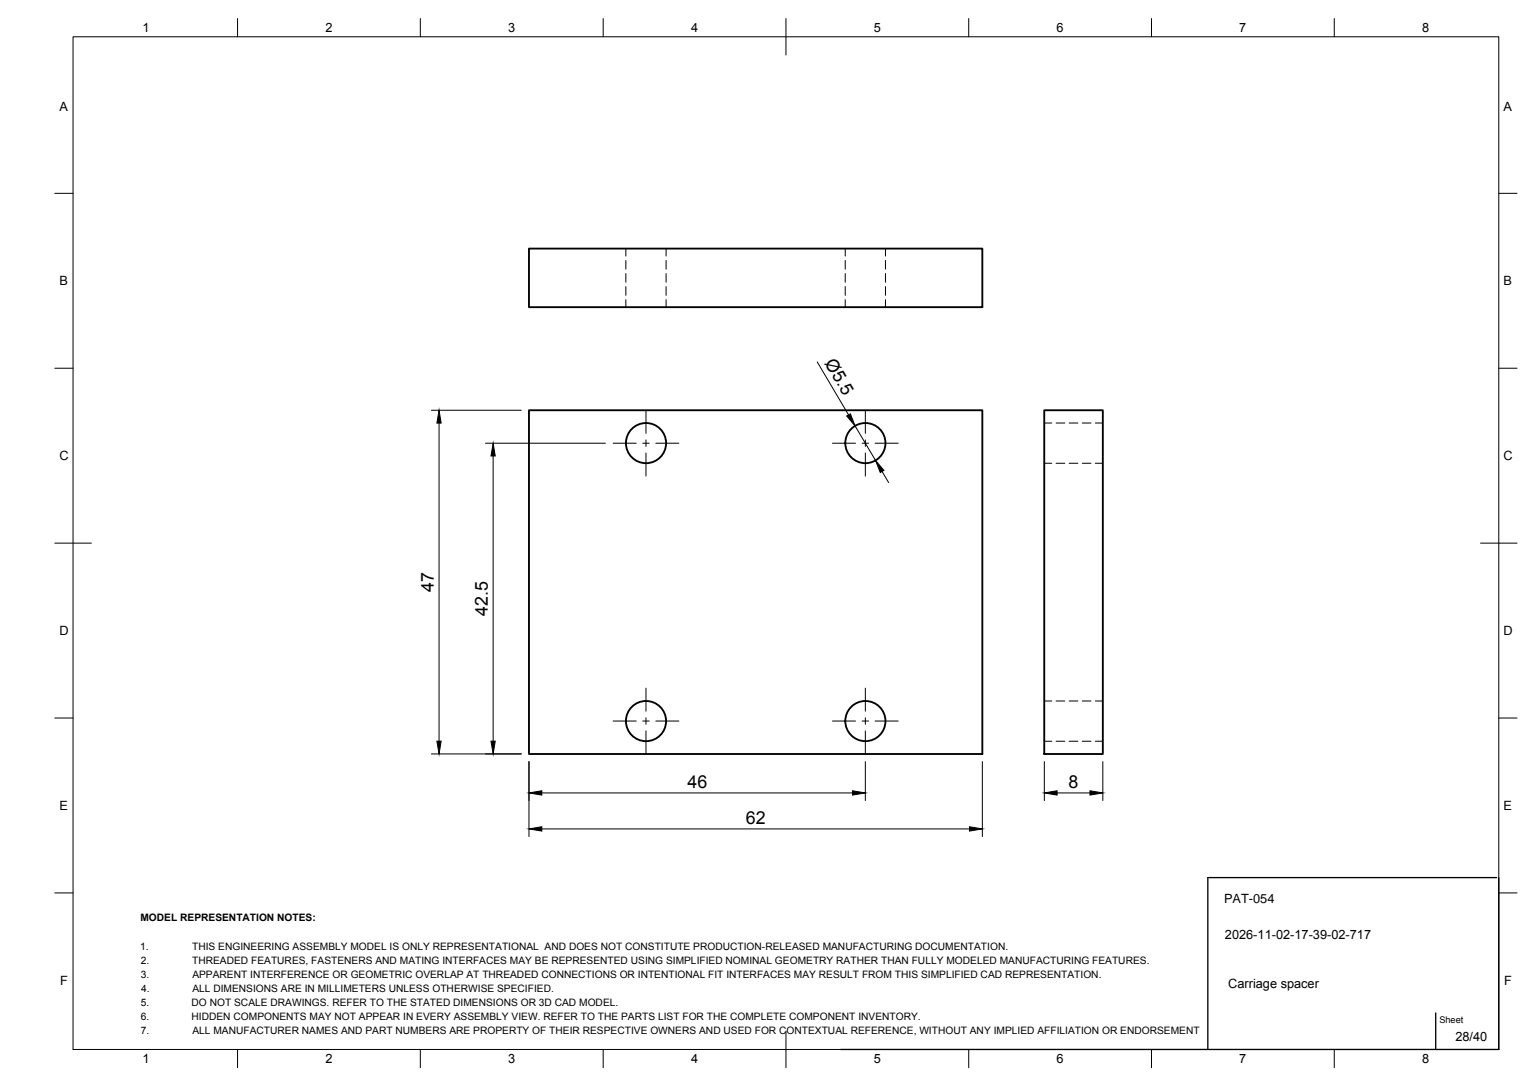
ISO-10303-21;
HEADER;
/* Generated by software containing ST-Developer
 * from STEP Tools, Inc. (www.steptools.com) 
 */

FILE_DESCRIPTION(
/* description */ ('PAT-054'),
/* implementation_level */ '2;1');

FILE_NAME(
/* name */ 'Carriage spacer.step',
/* time_stamp */ '2026-10-29T16:38:13-07:00',
/* author */ (''),
/* organization */ (''),
/* preprocessor_version */ 'ST-DEVELOPER v20.2',
/* originating_system */ 'Autodesk Translation Framework v15.17.0.0',
/* authorisation */ '');

FILE_SCHEMA (('AUTOMOTIVE_DESIGN { 1 0 10303 214 3 1 1 }'));
ENDSEC;

DATA;
#10=MECHANICAL_DESIGN_GEOMETRIC_PRESENTATION_REPRESENTATION('',(#937),#33981);
#834=SHAPE_REPRESENTATION_RELATIONSHIP('SRR','None',#34210,#878);
#878=ADVANCED_BREP_SHAPE_REPRESENTATION('',(#995),#33958);
#937=STYLED_ITEM('',(#34510),#995);
#995=MANIFOLD_SOLID_BREP('Body1',#13049);
#1152=FACE_BOUND('',#2777,.T.);
#1153=FACE_BOUND('',#2778,.T.);
#1154=FACE_BOUND('',#2779,.T.);
#1155=FACE_BOUND('',#2780,.T.);
#1156=FACE_BOUND('',#2782,.T.);
#1157=FACE_BOUND('',#2783,.T.);
#1158=FACE_BOUND('',#2784,.T.);
#1159=FACE_BOUND('',#2785,.T.);
#1412=PLANE('',#14249);
#1413=PLANE('',#14250);
#1414=PLANE('',#14251);
#1415=PLANE('',#14252);
#1416=PLANE('',#14253);
#1417=PLANE('',#14254);
#1905=FACE_OUTER_BOUND('',#2768,.T.);
#1906=FACE_OUTER_BOUND('',#2769,.T.);
#1907=FACE_OUTER_BOUND('',#2770,.T.);
#1908=FACE_OUTER_BOUND('',#2771,.T.);
#1909=FACE_OUTER_BOUND('',#2772,.T.);
#1910=FACE_OUTER_BOUND('',#2773,.T.);
#1911=FACE_OUTER_BOUND('',#2774,.T.);
#1912=FACE_OUTER_BOUND('',#2775,.T.);
#1913=FACE_OUTER_BOUND('',#2776,.T.);
#1914=FACE_OUTER_BOUND('',#2781,.T.);
#2768=EDGE_LOOP('',(#10037,#10038,#10039,#10040));
#2769=EDGE_LOOP('',(#10041,#10042,#10043,#10044));
#2770=EDGE_LOOP('',(#10045,#10046,#10047,#10048));
#2771=EDGE_LOOP('',(#10049,#10050,#10051,#10052));
#2772=EDGE_LOOP('',(#10053,#10054,#10055,#10056));
#2773=EDGE_LOOP('',(#10057,#10058,#10059,#10060));
#2774=EDGE_LOOP('',(#10061,#10062,#10063,#10064));
#2775=EDGE_LOOP('',(#10065,#10066,#10067,#10068));
#2776=EDGE_LOOP('',(#10069,#10070,#10071,#10072));
#2777=EDGE_LOOP('',(#10073));
#2778=EDGE_LOOP('',(#10074));
#2779=EDGE_LOOP('',(#10075));
#2780=EDGE_LOOP('',(#10076));
#2781=EDGE_LOOP('',(#10077,#10078,#10079,#10080));
#2782=EDGE_LOOP('',(#10081));
#2783=EDGE_LOOP('',(#10082));
#2784=EDGE_LOOP('',(#10083));
#2785=EDGE_LOOP('',(#10084));
#3670=LINE('',#20797,#4604);
#3671=LINE('',#20803,#4605);
#3672=LINE('',#20809,#4606);
#3673=LINE('',#20815,#4607);
#3674=LINE('',#20820,#4608);
#3675=LINE('',#20822,#4609);
#3676=LINE('',#20824,#4610);
#3677=LINE('',#20825,#4611);
#3678=LINE('',#20828,#4612);
#3679=LINE('',#20830,#4613);
#3680=LINE('',#20831,#4614);
#3681=LINE('',#20834,#4615);
#3682=LINE('',#20836,#4616);
#3683=LINE('',#20837,#4617);
#3684=LINE('',#20839,#4618);
#3685=LINE('',#20840,#4619);
#4604=VECTOR('',#16683,0.275);
#4605=VECTOR('',#16690,0.275);
#4606=VECTOR('',#16697,0.275);
#4607=VECTOR('',#16704,0.275);
#4608=VECTOR('',#16709,1.);
#4609=VECTOR('',#16710,1.);
#4610=VECTOR('',#16711,1.);
#4611=VECTOR('',#16712,1.);
#4612=VECTOR('',#16715,1.);
#4613=VECTOR('',#16716,1.);
#4614=VECTOR('',#16717,1.);
#4615=VECTOR('',#16720,1.);
#4616=VECTOR('',#16721,1.);
#4617=VECTOR('',#16722,1.);
#4618=VECTOR('',#16725,1.);
#4619=VECTOR('',#16726,1.);
#5412=CIRCLE('',#14238,0.275);
#5413=CIRCLE('',#14239,0.275);
#5414=CIRCLE('',#14241,0.275);
#5415=CIRCLE('',#14242,0.275);
#5416=CIRCLE('',#14244,0.275);
#5417=CIRCLE('',#14245,0.275);
#5418=CIRCLE('',#14247,0.275);
#5419=CIRCLE('',#14248,0.275);
#6102=VERTEX_POINT('',#20794);
#6103=VERTEX_POINT('',#20796);
#6104=VERTEX_POINT('',#20800);
#6105=VERTEX_POINT('',#20802);
#6106=VERTEX_POINT('',#20806);
#6107=VERTEX_POINT('',#20808);
#6108=VERTEX_POINT('',#20812);
#6109=VERTEX_POINT('',#20814);
#6110=VERTEX_POINT('',#20818);
#6111=VERTEX_POINT('',#20819);
#6112=VERTEX_POINT('',#20821);
#6113=VERTEX_POINT('',#20823);
#6114=VERTEX_POINT('',#20827);
#6115=VERTEX_POINT('',#20829);
#6116=VERTEX_POINT('',#20833);
#6117=VERTEX_POINT('',#20835);
#7518=EDGE_CURVE('',#6102,#6102,#5412,.T.);
#7519=EDGE_CURVE('',#6102,#6103,#3670,.T.);
#7520=EDGE_CURVE('',#6103,#6103,#5413,.T.);
#7521=EDGE_CURVE('',#6104,#6104,#5414,.T.);
#7522=EDGE_CURVE('',#6104,#6105,#3671,.T.);
#7523=EDGE_CURVE('',#6105,#6105,#5415,.T.);
#7524=EDGE_CURVE('',#6106,#6106,#5416,.T.);
#7525=EDGE_CURVE('',#6106,#6107,#3672,.T.);
#7526=EDGE_CURVE('',#6107,#6107,#5417,.T.);
#7527=EDGE_CURVE('',#6108,#6108,#5418,.T.);
#7528=EDGE_CURVE('',#6108,#6109,#3673,.T.);
#7529=EDGE_CURVE('',#6109,#6109,#5419,.T.);
#7530=EDGE_CURVE('',#6110,#6111,#3674,.T.);
#7531=EDGE_CURVE('',#6111,#6112,#3675,.T.);
#7532=EDGE_CURVE('',#6113,#6112,#3676,.T.);
#7533=EDGE_CURVE('',#6110,#6113,#3677,.T.);
#7534=EDGE_CURVE('',#6114,#6110,#3678,.T.);
#7535=EDGE_CURVE('',#6115,#6113,#3679,.T.);
#7536=EDGE_CURVE('',#6114,#6115,#3680,.T.);
#7537=EDGE_CURVE('',#6116,#6114,#3681,.T.);
#7538=EDGE_CURVE('',#6117,#6115,#3682,.T.);
#7539=EDGE_CURVE('',#6116,#6117,#3683,.T.);
#7540=EDGE_CURVE('',#6111,#6116,#3684,.T.);
#7541=EDGE_CURVE('',#6112,#6117,#3685,.T.);
#10037=ORIENTED_EDGE('',*,*,#7518,.F.);
#10038=ORIENTED_EDGE('',*,*,#7519,.T.);
#10039=ORIENTED_EDGE('',*,*,#7520,.F.);
#10040=ORIENTED_EDGE('',*,*,#7519,.F.);
#10041=ORIENTED_EDGE('',*,*,#7521,.F.);
#10042=ORIENTED_EDGE('',*,*,#7522,.T.);
#10043=ORIENTED_EDGE('',*,*,#7523,.F.);
#10044=ORIENTED_EDGE('',*,*,#7522,.F.);
#10045=ORIENTED_EDGE('',*,*,#7524,.F.);
#10046=ORIENTED_EDGE('',*,*,#7525,.T.);
#10047=ORIENTED_EDGE('',*,*,#7526,.F.);
#10048=ORIENTED_EDGE('',*,*,#7525,.F.);
#10049=ORIENTED_EDGE('',*,*,#7527,.F.);
#10050=ORIENTED_EDGE('',*,*,#7528,.T.);
#10051=ORIENTED_EDGE('',*,*,#7529,.F.);
#10052=ORIENTED_EDGE('',*,*,#7528,.F.);
#10053=ORIENTED_EDGE('',*,*,#7530,.T.);
#10054=ORIENTED_EDGE('',*,*,#7531,.T.);
#10055=ORIENTED_EDGE('',*,*,#7532,.F.);
#10056=ORIENTED_EDGE('',*,*,#7533,.F.);
#10057=ORIENTED_EDGE('',*,*,#7534,.T.);
#10058=ORIENTED_EDGE('',*,*,#7533,.T.);
#10059=ORIENTED_EDGE('',*,*,#7535,.F.);
#10060=ORIENTED_EDGE('',*,*,#7536,.F.);
#10061=ORIENTED_EDGE('',*,*,#7537,.T.);
#10062=ORIENTED_EDGE('',*,*,#7536,.T.);
#10063=ORIENTED_EDGE('',*,*,#7538,.F.);
#10064=ORIENTED_EDGE('',*,*,#7539,.F.);
#10065=ORIENTED_EDGE('',*,*,#7540,.T.);
#10066=ORIENTED_EDGE('',*,*,#7539,.T.);
#10067=ORIENTED_EDGE('',*,*,#7541,.F.);
#10068=ORIENTED_EDGE('',*,*,#7531,.F.);
#10069=ORIENTED_EDGE('',*,*,#7541,.T.);
#10070=ORIENTED_EDGE('',*,*,#7538,.T.);
#10071=ORIENTED_EDGE('',*,*,#7535,.T.);
#10072=ORIENTED_EDGE('',*,*,#7532,.T.);
#10073=ORIENTED_EDGE('',*,*,#7520,.T.);
#10074=ORIENTED_EDGE('',*,*,#7523,.T.);
#10075=ORIENTED_EDGE('',*,*,#7526,.T.);
#10076=ORIENTED_EDGE('',*,*,#7529,.T.);
#10077=ORIENTED_EDGE('',*,*,#7540,.F.);
#10078=ORIENTED_EDGE('',*,*,#7530,.F.);
#10079=ORIENTED_EDGE('',*,*,#7534,.F.);
#10080=ORIENTED_EDGE('',*,*,#7537,.F.);
#10081=ORIENTED_EDGE('',*,*,#7518,.T.);
#10082=ORIENTED_EDGE('',*,*,#7521,.T.);
#10083=ORIENTED_EDGE('',*,*,#7524,.T.);
#10084=ORIENTED_EDGE('',*,*,#7527,.T.);
#12079=CYLINDRICAL_SURFACE('',#14237,0.275);
#12080=CYLINDRICAL_SURFACE('',#14240,0.275);
#12081=CYLINDRICAL_SURFACE('',#14243,0.275);
#12082=CYLINDRICAL_SURFACE('',#14246,0.275);
#12617=ADVANCED_FACE('',(#1905),#12079,.F.);
#12618=ADVANCED_FACE('',(#1906),#12080,.F.);
#12619=ADVANCED_FACE('',(#1907),#12081,.F.);
#12620=ADVANCED_FACE('',(#1908),#12082,.F.);
#12621=ADVANCED_FACE('',(#1909),#1412,.T.);
#12622=ADVANCED_FACE('',(#1910),#1413,.T.);
#12623=ADVANCED_FACE('',(#1911),#1414,.T.);
#12624=ADVANCED_FACE('',(#1912),#1415,.T.);
#12625=ADVANCED_FACE('',(#1913,#1152,#1153,#1154,#1155),#1416,.T.);
#12626=ADVANCED_FACE('',(#1914,#1156,#1157,#1158,#1159),#1417,.F.);
#13049=CLOSED_SHELL('',(#12617,#12618,#12619,#12620,#12621,#12622,#12623,
#12624,#12625,#12626));
#14236=AXIS2_PLACEMENT_3D('',#20792,#16677,#16678);
#14237=AXIS2_PLACEMENT_3D('',#20793,#16679,#16680);
#14238=AXIS2_PLACEMENT_3D('',#20795,#16681,#16682);
#14239=AXIS2_PLACEMENT_3D('',#20798,#16684,#16685);
#14240=AXIS2_PLACEMENT_3D('',#20799,#16686,#16687);
#14241=AXIS2_PLACEMENT_3D('',#20801,#16688,#16689);
#14242=AXIS2_PLACEMENT_3D('',#20804,#16691,#16692);
#14243=AXIS2_PLACEMENT_3D('',#20805,#16693,#16694);
#14244=AXIS2_PLACEMENT_3D('',#20807,#16695,#16696);
#14245=AXIS2_PLACEMENT_3D('',#20810,#16698,#16699);
#14246=AXIS2_PLACEMENT_3D('',#20811,#16700,#16701);
#14247=AXIS2_PLACEMENT_3D('',#20813,#16702,#16703);
#14248=AXIS2_PLACEMENT_3D('',#20816,#16705,#16706);
#14249=AXIS2_PLACEMENT_3D('',#20817,#16707,#16708);
#14250=AXIS2_PLACEMENT_3D('',#20826,#16713,#16714);
#14251=AXIS2_PLACEMENT_3D('',#20832,#16718,#16719);
#14252=AXIS2_PLACEMENT_3D('',#20838,#16723,#16724);
#14253=AXIS2_PLACEMENT_3D('',#20841,#16727,#16728);
#14254=AXIS2_PLACEMENT_3D('',#20842,#16729,#16730);
#16677=DIRECTION('axis',(0.,0.,1.));
#16678=DIRECTION('refdir',(1.,0.,0.));
#16679=DIRECTION('center_axis',(0.,0.,1.));
#16680=DIRECTION('ref_axis',(1.,0.,0.));
#16681=DIRECTION('center_axis',(0.,0.,1.));
#16682=DIRECTION('ref_axis',(1.,0.,0.));
#16683=DIRECTION('',(0.,0.,1.));
#16684=DIRECTION('center_axis',(0.,0.,-1.));
#16685=DIRECTION('ref_axis',(1.,0.,0.));
#16686=DIRECTION('center_axis',(0.,0.,1.));
#16687=DIRECTION('ref_axis',(1.,0.,0.));
#16688=DIRECTION('center_axis',(0.,0.,1.));
#16689=DIRECTION('ref_axis',(1.,0.,0.));
#16690=DIRECTION('',(0.,0.,1.));
#16691=DIRECTION('center_axis',(0.,0.,-1.));
#16692=DIRECTION('ref_axis',(1.,0.,0.));
#16693=DIRECTION('center_axis',(0.,0.,1.));
#16694=DIRECTION('ref_axis',(1.,0.,0.));
#16695=DIRECTION('center_axis',(0.,0.,1.));
#16696=DIRECTION('ref_axis',(1.,0.,0.));
#16697=DIRECTION('',(0.,0.,1.));
#16698=DIRECTION('center_axis',(0.,0.,-1.));
#16699=DIRECTION('ref_axis',(1.,0.,0.));
#16700=DIRECTION('center_axis',(0.,0.,1.));
#16701=DIRECTION('ref_axis',(1.,0.,0.));
#16702=DIRECTION('center_axis',(0.,0.,1.));
#16703=DIRECTION('ref_axis',(1.,0.,0.));
#16704=DIRECTION('',(0.,0.,1.));
#16705=DIRECTION('center_axis',(0.,0.,-1.));
#16706=DIRECTION('ref_axis',(1.,0.,0.));
#16707=DIRECTION('center_axis',(0.,1.,0.));
#16708=DIRECTION('ref_axis',(-1.,0.,0.));
#16709=DIRECTION('',(-1.,0.,0.));
#16710=DIRECTION('',(0.,0.,1.));
#16711=DIRECTION('',(-1.,0.,0.));
#16712=DIRECTION('',(0.,0.,1.));
#16713=DIRECTION('center_axis',(1.,0.,0.));
#16714=DIRECTION('ref_axis',(0.,1.,0.));
#16715=DIRECTION('',(0.,1.,0.));
#16716=DIRECTION('',(0.,1.,0.));
#16717=DIRECTION('',(0.,0.,1.));
#16718=DIRECTION('center_axis',(0.,-1.,0.));
#16719=DIRECTION('ref_axis',(1.,0.,0.));
#16720=DIRECTION('',(1.,0.,0.));
#16721=DIRECTION('',(1.,0.,0.));
#16722=DIRECTION('',(0.,0.,1.));
#16723=DIRECTION('center_axis',(-1.,0.,0.));
#16724=DIRECTION('ref_axis',(0.,-1.,0.));
#16725=DIRECTION('',(0.,-1.,0.));
#16726=DIRECTION('',(0.,-1.,0.));
#16727=DIRECTION('center_axis',(0.,0.,1.));
#16728=DIRECTION('ref_axis',(1.,0.,0.));
#16729=DIRECTION('center_axis',(0.,0.,1.));
#16730=DIRECTION('ref_axis',(1.,0.,0.));
#20792=CARTESIAN_POINT('',(0.,0.,0.));
#20793=CARTESIAN_POINT('Origin',(15.,-7.9,5.1));
#20794=CARTESIAN_POINT('',(14.725,-7.9,5.2));
#20795=CARTESIAN_POINT('Origin',(15.,-7.9,5.2));
#20796=CARTESIAN_POINT('',(14.725,-7.9,6.));
#20797=CARTESIAN_POINT('',(14.725,-7.9,5.1));
#20798=CARTESIAN_POINT('Origin',(15.,-7.9,6.));
#20799=CARTESIAN_POINT('Origin',(12.,-4.1,5.1));
#20800=CARTESIAN_POINT('',(11.725,-4.1,5.2));
#20801=CARTESIAN_POINT('Origin',(12.,-4.1,5.2));
#20802=CARTESIAN_POINT('',(11.725,-4.1,6.));
#20803=CARTESIAN_POINT('',(11.725,-4.1,5.1));
#20804=CARTESIAN_POINT('Origin',(12.,-4.1,6.));
#20805=CARTESIAN_POINT('Origin',(12.,-7.9,5.1));
#20806=CARTESIAN_POINT('',(11.725,-7.9,5.2));
#20807=CARTESIAN_POINT('Origin',(12.,-7.9,5.2));
#20808=CARTESIAN_POINT('',(11.725,-7.9,6.));
#20809=CARTESIAN_POINT('',(11.725,-7.9,5.1));
#20810=CARTESIAN_POINT('Origin',(12.,-7.9,6.));
#20811=CARTESIAN_POINT('Origin',(15.,-4.1,5.1));
#20812=CARTESIAN_POINT('',(14.725,-4.1,5.2));
#20813=CARTESIAN_POINT('Origin',(15.,-4.1,5.2));
#20814=CARTESIAN_POINT('',(14.725,-4.1,6.));
#20815=CARTESIAN_POINT('',(14.725,-4.1,5.1));
#20816=CARTESIAN_POINT('Origin',(15.,-4.1,6.));
#20817=CARTESIAN_POINT('Origin',(16.6,-3.65,5.2));
#20818=CARTESIAN_POINT('',(16.6,-3.65,5.2));
#20819=CARTESIAN_POINT('',(10.4,-3.65,5.2));
#20820=CARTESIAN_POINT('',(16.6,-3.65,5.2));
#20821=CARTESIAN_POINT('',(10.4,-3.65,6.));
#20822=CARTESIAN_POINT('',(10.4,-3.65,5.2));
#20823=CARTESIAN_POINT('',(16.6,-3.65,6.));
#20824=CARTESIAN_POINT('',(16.6,-3.65,6.));
#20825=CARTESIAN_POINT('',(16.6,-3.65,5.2));
#20826=CARTESIAN_POINT('Origin',(16.6,-8.35,5.2));
#20827=CARTESIAN_POINT('',(16.6,-8.35,5.2));
#20828=CARTESIAN_POINT('',(16.6,-8.35,5.2));
#20829=CARTESIAN_POINT('',(16.6,-8.35,6.));
#20830=CARTESIAN_POINT('',(16.6,-8.35,6.));
#20831=CARTESIAN_POINT('',(16.6,-8.35,5.2));
#20832=CARTESIAN_POINT('Origin',(10.4,-8.35,5.2));
#20833=CARTESIAN_POINT('',(10.4,-8.35,5.2));
#20834=CARTESIAN_POINT('',(10.4,-8.35,5.2));
#20835=CARTESIAN_POINT('',(10.4,-8.35,6.));
#20836=CARTESIAN_POINT('',(10.4,-8.35,6.));
#20837=CARTESIAN_POINT('',(10.4,-8.35,5.2));
#20838=CARTESIAN_POINT('Origin',(10.4,-3.65,5.2));
#20839=CARTESIAN_POINT('',(10.4,-3.65,5.2));
#20840=CARTESIAN_POINT('',(10.4,-3.65,6.));
#20841=CARTESIAN_POINT('Origin',(13.5,-6.,6.));
#20842=CARTESIAN_POINT('Origin',(13.5,-6.,5.2));
#33906=UNCERTAINTY_MEASURE_WITH_UNIT(LENGTH_MEASURE(0.001),#33982,
'DISTANCE_ACCURACY_VALUE',
'Maximum model space distance between geometric entities at asserted c
onnectivities');
#33929=UNCERTAINTY_MEASURE_WITH_UNIT(LENGTH_MEASURE(0.001),#33982,
'DISTANCE_ACCURACY_VALUE',
'Maximum model space distance between geometric entities at asserted c
onnectivities');
#33958=(
GEOMETRIC_REPRESENTATION_CONTEXT(3)
GLOBAL_UNCERTAINTY_ASSIGNED_CONTEXT((#33906))
GLOBAL_UNIT_ASSIGNED_CONTEXT((#33982,#33984,#33985))
REPRESENTATION_CONTEXT('','3D')
);
#33981=(
GEOMETRIC_REPRESENTATION_CONTEXT(3)
GLOBAL_UNCERTAINTY_ASSIGNED_CONTEXT((#33929))
GLOBAL_UNIT_ASSIGNED_CONTEXT((#33982,#33984,#33985))
REPRESENTATION_CONTEXT('','3D')
);
#33982=(
LENGTH_UNIT()
NAMED_UNIT(*)
SI_UNIT(.CENTI.,.METRE.)
);
#33984=(
NAMED_UNIT(*)
PLANE_ANGLE_UNIT()
SI_UNIT($,.RADIAN.)
);
#33985=(
NAMED_UNIT(*)
SI_UNIT($,.STERADIAN.)
SOLID_ANGLE_UNIT()
);
#34014=SHAPE_DEFINITION_REPRESENTATION(#34075,#34210);
#34075=PRODUCT_DEFINITION_SHAPE('',$,#34262);
#34210=SHAPE_REPRESENTATION('',(#14236),#33958);
#34233=PRODUCT_DEFINITION_CONTEXT('part definition',#34388,'design');
#34262=PRODUCT_DEFINITION('Carriage spacer','Carriage spacer',#34313,#34233);
#34313=PRODUCT_DEFINITION_FORMATION('',$,#34418);
#34388=APPLICATION_CONTEXT(
'Core Data for Automotive Mechanical Design Process');
#34389=PRODUCT_CONTEXT('part definition',#34388,'mechanical');
#34418=PRODUCT('Carriage spacer','Carriage spacer','Carriage spacer',(#34389));
#34504=COLOUR_RGB('Sky Blue',0.24,0.69,0.87);
#34505=FILL_AREA_STYLE_COLOUR('',#34504);
#34506=FILL_AREA_STYLE('',(#34505));
#34507=SURFACE_STYLE_FILL_AREA(#34506);
#34508=SURFACE_SIDE_STYLE('',(#34507));
#34509=SURFACE_STYLE_USAGE(.BOTH.,#34508);
#34510=PRESENTATION_STYLE_ASSIGNMENT((#34509));
ENDSEC;
END-ISO-10303-21;
